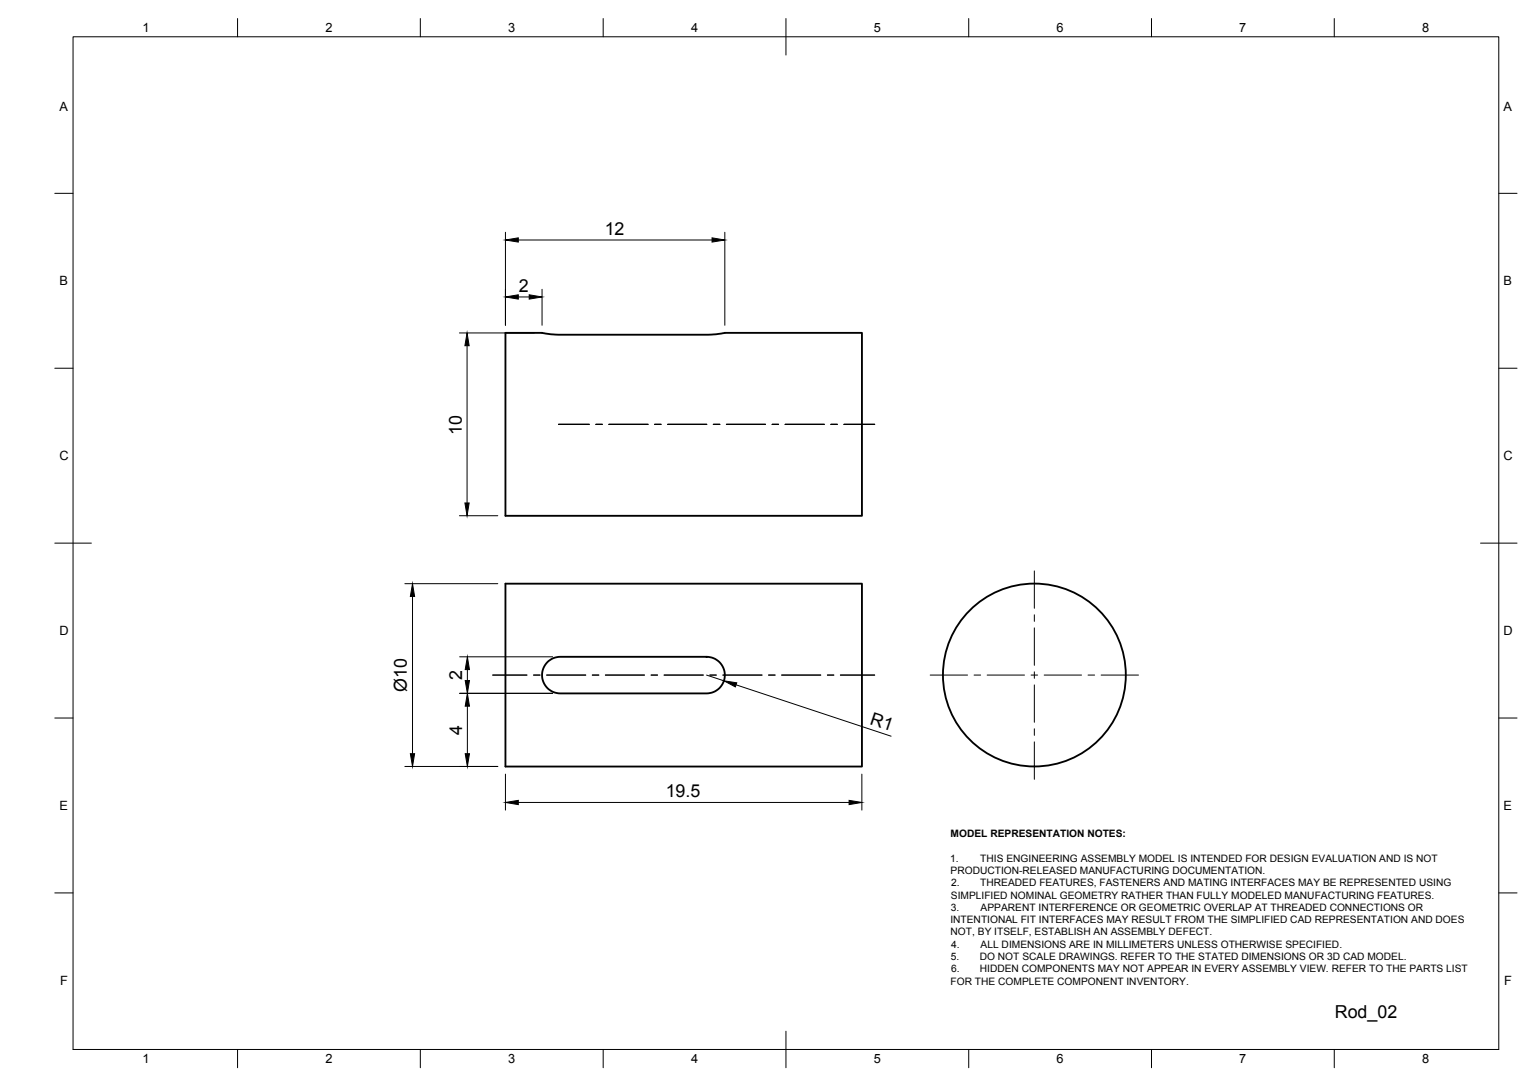
ISO-10303-21;
HEADER;
/* Generated by software containing ST-Developer
 * from STEP Tools, Inc. (www.steptools.com) 
 */

FILE_DESCRIPTION(
/* description */ (''),
/* implementation_level */ '2;1');

FILE_NAME(
/* name */ 'Rod_02.step',
/* time_stamp */ '2026-10-05T21:34:53-07:00',
/* author */ (''),
/* organization */ (''),
/* preprocessor_version */ 'ST-DEVELOPER v20.2',
/* originating_system */ 'Autodesk Translation Framework v15.15.0.0',
/* authorisation */ '');

FILE_SCHEMA (('AUTOMOTIVE_DESIGN { 1 0 10303 214 3 1 1 }'));
ENDSEC;

DATA;
#10=MECHANICAL_DESIGN_GEOMETRIC_PRESENTATION_REPRESENTATION('',(#71),#9822);
#53=SHAPE_REPRESENTATION_RELATIONSHIP('SRR','None',#9863,#62);
#62=ADVANCED_BREP_SHAPE_REPRESENTATION('',(#80),#9819);
#71=STYLED_ITEM('',(#9912),#80);
#80=MANIFOLD_SOLID_BREP('Body1',#3294);
#98=FACE_BOUND('',#637,.T.);
#155=B_SPLINE_CURVE_WITH_KNOTS('',3,(#9682,#9683,#9684,#9685,#9686,#9687,
#9688,#9689,#9690,#9691,#9692,#9693,#9694,#9695,#9696,#9697,#9698,#9699),
 .UNSPECIFIED.,.F.,.F.,(4,2,2,2,2,2,2,2,4),(-0.302227736861757,-0.264448211272738,
-0.226668685683718,-0.188891277057298,-0.151113868430879,-0.113336459804459,
-0.0755590511780388,-0.0377795255890194,0.),.UNSPECIFIED.);
#156=B_SPLINE_CURVE_WITH_KNOTS('',3,(#9712,#9713,#9714,#9715,#9716,#9717,
#9718,#9719,#9720,#9721,#9722,#9723,#9724,#9725,#9726,#9727,#9728,#9729),
 .UNSPECIFIED.,.F.,.F.,(4,2,2,2,2,2,2,2,4),(-0.604455473723515,-0.566675948134495,
-0.528896422545476,-0.491119013919056,-0.453341605292636,-0.415564196666216,
-0.377786788039796,-0.340007262450777,-0.302227736861757),.UNSPECIFIED.);
#252=PLANE('',#3684);
#253=PLANE('',#3687);
#254=PLANE('',#3689);
#255=PLANE('',#3691);
#256=PLANE('',#3695);
#430=FACE_OUTER_BOUND('',#630,.T.);
#431=FACE_OUTER_BOUND('',#631,.T.);
#432=FACE_OUTER_BOUND('',#632,.T.);
#433=FACE_OUTER_BOUND('',#633,.T.);
#434=FACE_OUTER_BOUND('',#634,.T.);
#435=FACE_OUTER_BOUND('',#635,.T.);
#436=FACE_OUTER_BOUND('',#636,.T.);
#437=FACE_OUTER_BOUND('',#638,.T.);
#630=EDGE_LOOP('',(#2948,#2949,#2950,#2951));
#631=EDGE_LOOP('',(#2952,#2953,#2954,#2955));
#632=EDGE_LOOP('',(#2956,#2957,#2958,#2959));
#633=EDGE_LOOP('',(#2960,#2961,#2962,#2963));
#634=EDGE_LOOP('',(#2964,#2965,#2966,#2967));
#635=EDGE_LOOP('',(#2968));
#636=EDGE_LOOP('',(#2969,#2970,#2971,#2972));
#637=EDGE_LOOP('',(#2973,#2974,#2975,#2976));
#638=EDGE_LOOP('',(#2977));
#885=LINE('',#9674,#1144);
#886=LINE('',#9676,#1145);
#887=LINE('',#9678,#1146);
#888=LINE('',#9679,#1147);
#889=LINE('',#9701,#1148);
#890=LINE('',#9705,#1149);
#891=LINE('',#9709,#1150);
#892=LINE('',#9710,#1151);
#893=LINE('',#9735,#1152);
#1144=VECTOR('',#4537,10.);
#1145=VECTOR('',#4538,10.);
#1146=VECTOR('',#4539,10.);
#1147=VECTOR('',#4540,10.);
#1148=VECTOR('',#4543,10.);
#1149=VECTOR('',#4548,10.);
#1150=VECTOR('',#4553,10.);
#1151=VECTOR('',#4554,10.);
#1152=VECTOR('',#4563,5.);
#1307=CIRCLE('',#3686,1.);
#1308=CIRCLE('',#3688,1.);
#1309=CIRCLE('',#3692,5.);
#1310=CIRCLE('',#3694,5.);
#1599=VERTEX_POINT('',#9672);
#1600=VERTEX_POINT('',#9673);
#1601=VERTEX_POINT('',#9675);
#1602=VERTEX_POINT('',#9677);
#1603=VERTEX_POINT('',#9681);
#1604=VERTEX_POINT('',#9700);
#1605=VERTEX_POINT('',#9704);
#1606=VERTEX_POINT('',#9708);
#1607=VERTEX_POINT('',#9731);
#1608=VERTEX_POINT('',#9734);
#2053=EDGE_CURVE('',#1599,#1600,#885,.T.);
#2054=EDGE_CURVE('',#1601,#1600,#886,.T.);
#2055=EDGE_CURVE('',#1601,#1602,#887,.T.);
#2056=EDGE_CURVE('',#1602,#1599,#888,.T.);
#2057=EDGE_CURVE('',#1600,#1603,#155,.T.);
#2058=EDGE_CURVE('',#1604,#1603,#889,.T.);
#2059=EDGE_CURVE('',#1604,#1601,#1307,.T.);
#2060=EDGE_CURVE('',#1605,#1604,#890,.T.);
#2061=EDGE_CURVE('',#1602,#1605,#1308,.T.);
#2062=EDGE_CURVE('',#1603,#1606,#891,.T.);
#2063=EDGE_CURVE('',#1605,#1606,#892,.T.);
#2064=EDGE_CURVE('',#1606,#1599,#156,.T.);
#2065=EDGE_CURVE('',#1607,#1607,#1309,.T.);
#2066=EDGE_CURVE('',#1607,#1608,#893,.T.);
#2067=EDGE_CURVE('',#1608,#1608,#1310,.T.);
#2948=ORIENTED_EDGE('',*,*,#2053,.T.);
#2949=ORIENTED_EDGE('',*,*,#2054,.F.);
#2950=ORIENTED_EDGE('',*,*,#2055,.T.);
#2951=ORIENTED_EDGE('',*,*,#2056,.T.);
#2952=ORIENTED_EDGE('',*,*,#2057,.T.);
#2953=ORIENTED_EDGE('',*,*,#2058,.F.);
#2954=ORIENTED_EDGE('',*,*,#2059,.T.);
#2955=ORIENTED_EDGE('',*,*,#2054,.T.);
#2956=ORIENTED_EDGE('',*,*,#2059,.F.);
#2957=ORIENTED_EDGE('',*,*,#2060,.F.);
#2958=ORIENTED_EDGE('',*,*,#2061,.F.);
#2959=ORIENTED_EDGE('',*,*,#2055,.F.);
#2960=ORIENTED_EDGE('',*,*,#2062,.T.);
#2961=ORIENTED_EDGE('',*,*,#2063,.F.);
#2962=ORIENTED_EDGE('',*,*,#2060,.T.);
#2963=ORIENTED_EDGE('',*,*,#2058,.T.);
#2964=ORIENTED_EDGE('',*,*,#2064,.T.);
#2965=ORIENTED_EDGE('',*,*,#2056,.F.);
#2966=ORIENTED_EDGE('',*,*,#2061,.T.);
#2967=ORIENTED_EDGE('',*,*,#2063,.T.);
#2968=ORIENTED_EDGE('',*,*,#2065,.F.);
#2969=ORIENTED_EDGE('',*,*,#2065,.T.);
#2970=ORIENTED_EDGE('',*,*,#2066,.T.);
#2971=ORIENTED_EDGE('',*,*,#2067,.T.);
#2972=ORIENTED_EDGE('',*,*,#2066,.F.);
#2973=ORIENTED_EDGE('',*,*,#2062,.F.);
#2974=ORIENTED_EDGE('',*,*,#2057,.F.);
#2975=ORIENTED_EDGE('',*,*,#2053,.F.);
#2976=ORIENTED_EDGE('',*,*,#2064,.F.);
#2977=ORIENTED_EDGE('',*,*,#2067,.F.);
#3096=CYLINDRICAL_SURFACE('',#3685,1.);
#3097=CYLINDRICAL_SURFACE('',#3690,1.);
#3098=CYLINDRICAL_SURFACE('',#3693,5.);
#3268=ADVANCED_FACE('',(#430),#252,.T.);
#3269=ADVANCED_FACE('',(#431),#3096,.F.);
#3270=ADVANCED_FACE('',(#432),#253,.T.);
#3271=ADVANCED_FACE('',(#433),#254,.T.);
#3272=ADVANCED_FACE('',(#434),#3097,.F.);
#3273=ADVANCED_FACE('',(#435),#255,.T.);
#3274=ADVANCED_FACE('',(#436,#98),#3098,.T.);
#3275=ADVANCED_FACE('',(#437),#256,.F.);
#3294=CLOSED_SHELL('',(#3268,#3269,#3270,#3271,#3272,#3273,#3274,#3275));
#3683=AXIS2_PLACEMENT_3D('',#9670,#4533,#4534);
#3684=AXIS2_PLACEMENT_3D('',#9671,#4535,#4536);
#3685=AXIS2_PLACEMENT_3D('',#9680,#4541,#4542);
#3686=AXIS2_PLACEMENT_3D('',#9702,#4544,#4545);
#3687=AXIS2_PLACEMENT_3D('',#9703,#4546,#4547);
#3688=AXIS2_PLACEMENT_3D('',#9706,#4549,#4550);
#3689=AXIS2_PLACEMENT_3D('',#9707,#4551,#4552);
#3690=AXIS2_PLACEMENT_3D('',#9711,#4555,#4556);
#3691=AXIS2_PLACEMENT_3D('',#9730,#4557,#4558);
#3692=AXIS2_PLACEMENT_3D('',#9732,#4559,#4560);
#3693=AXIS2_PLACEMENT_3D('',#9733,#4561,#4562);
#3694=AXIS2_PLACEMENT_3D('',#9736,#4564,#4565);
#3695=AXIS2_PLACEMENT_3D('',#9737,#4566,#4567);
#4533=DIRECTION('axis',(0.,0.,1.));
#4534=DIRECTION('refdir',(1.,0.,0.));
#4535=DIRECTION('center_axis',(-1.,0.,0.));
#4536=DIRECTION('ref_axis',(0.,0.,-1.));
#4537=DIRECTION('',(0.,0.,1.));
#4538=DIRECTION('',(0.,-1.,0.));
#4539=DIRECTION('',(0.,0.,-1.));
#4540=DIRECTION('',(0.,-1.,0.));
#4541=DIRECTION('center_axis',(0.,1.,0.));
#4542=DIRECTION('ref_axis',(1.,0.,0.));
#4543=DIRECTION('',(0.,-1.,0.));
#4544=DIRECTION('center_axis',(0.,1.,0.));
#4545=DIRECTION('ref_axis',(1.,0.,0.));
#4546=DIRECTION('center_axis',(0.,-1.,0.));
#4547=DIRECTION('ref_axis',(1.,0.,0.));
#4548=DIRECTION('',(0.,0.,1.));
#4549=DIRECTION('center_axis',(0.,1.,0.));
#4550=DIRECTION('ref_axis',(-1.,0.,0.));
#4551=DIRECTION('center_axis',(1.,0.,0.));
#4552=DIRECTION('ref_axis',(0.,0.,1.));
#4553=DIRECTION('',(0.,0.,-1.));
#4554=DIRECTION('',(0.,-1.,0.));
#4555=DIRECTION('center_axis',(0.,1.,0.));
#4556=DIRECTION('ref_axis',(-1.,0.,0.));
#4557=DIRECTION('center_axis',(0.,0.,1.));
#4558=DIRECTION('ref_axis',(-1.,0.,0.));
#4559=DIRECTION('center_axis',(0.,0.,-1.));
#4560=DIRECTION('ref_axis',(-1.,0.,0.));
#4561=DIRECTION('center_axis',(0.,0.,1.));
#4562=DIRECTION('ref_axis',(-1.,0.,0.));
#4563=DIRECTION('',(0.,0.,-1.));
#4564=DIRECTION('center_axis',(0.,0.,1.));
#4565=DIRECTION('ref_axis',(-1.,0.,0.));
#4566=DIRECTION('center_axis',(0.,0.,1.));
#4567=DIRECTION('ref_axis',(-1.,0.,0.));
#9670=CARTESIAN_POINT('',(0.,0.,0.));
#9671=CARTESIAN_POINT('Origin',(1.,0.,-6.5));
#9672=CARTESIAN_POINT('',(1.,-4.89897948556636,-14.5));
#9673=CARTESIAN_POINT('',(1.,-4.89897948556636,-6.5));
#9674=CARTESIAN_POINT('',(1.,-4.89897948556636,-12.));
#9675=CARTESIAN_POINT('',(1.,-4.,-6.5));
#9676=CARTESIAN_POINT('',(1.,0.,-6.5));
#9677=CARTESIAN_POINT('',(1.,-4.,-14.5));
#9678=CARTESIAN_POINT('',(1.,-4.,-8.5));
#9679=CARTESIAN_POINT('',(1.,0.,-14.5));
#9680=CARTESIAN_POINT('Origin',(0.,0.,-6.5));
#9681=CARTESIAN_POINT('',(-1.,-4.89897948556636,-6.5));
#9682=CARTESIAN_POINT('Ctrl Pts',(1.,-4.89897948556636,-6.5));
#9683=CARTESIAN_POINT('Ctrl Pts',(1.,-4.89897948556636,-6.3740682480366));
#9684=CARTESIAN_POINT('Ctrl Pts',(0.974762796248615,-4.90433876618447,-6.23998222283811));
#9685=CARTESIAN_POINT('Ctrl Pts',(0.872605417648384,-4.92354150792771,-5.99370799496995));
#9686=CARTESIAN_POINT('Ctrl Pts',(0.795703102192088,-4.93709085101933,-5.88148953981899));
#9687=CARTESIAN_POINT('Ctrl Pts',(0.618515424645094,-4.96240337638318,-5.704301862272));
#9688=CARTESIAN_POINT('Ctrl Pts',(0.506294861197626,-4.97583347151864,-5.62739565845524));
#9689=CARTESIAN_POINT('Ctrl Pts',(0.260013306081865,-4.99476188647081,-5.52523545776417));
#9690=CARTESIAN_POINT('Ctrl Pts',(0.125924695421399,-5.,-5.5));
#9691=CARTESIAN_POINT('Ctrl Pts',(-0.1259246954214,-5.,-5.5));
#9692=CARTESIAN_POINT('Ctrl Pts',(-0.260013306081865,-4.99476188647081,
-5.52523545776417));
#9693=CARTESIAN_POINT('Ctrl Pts',(-0.506294861197626,-4.97583347151864,
-5.62739565845524));
#9694=CARTESIAN_POINT('Ctrl Pts',(-0.618515424645094,-4.96240337638318,
-5.704301862272));
#9695=CARTESIAN_POINT('Ctrl Pts',(-0.795703102192089,-4.93709085101933,
-5.88148953981899));
#9696=CARTESIAN_POINT('Ctrl Pts',(-0.872605417648382,-4.92354150792771,
-5.99370799496995));
#9697=CARTESIAN_POINT('Ctrl Pts',(-0.974762796248614,-4.90433876618447,
-6.23998222283811));
#9698=CARTESIAN_POINT('Ctrl Pts',(-1.,-4.89897948556636,-6.3740682480366));
#9699=CARTESIAN_POINT('Ctrl Pts',(-1.,-4.89897948556636,-6.5));
#9700=CARTESIAN_POINT('',(-1.,-4.,-6.5));
#9701=CARTESIAN_POINT('',(-1.,0.,-6.5));
#9702=CARTESIAN_POINT('Origin',(0.,-4.,-6.5));
#9703=CARTESIAN_POINT('Origin',(0.,-4.,-10.5));
#9704=CARTESIAN_POINT('',(-1.,-4.,-14.5));
#9705=CARTESIAN_POINT('',(-1.,-4.,-12.5));
#9706=CARTESIAN_POINT('Origin',(0.,-4.,-14.5));
#9707=CARTESIAN_POINT('Origin',(-1.,0.,-14.5));
#9708=CARTESIAN_POINT('',(-1.,-4.89897948556636,-14.5));
#9709=CARTESIAN_POINT('',(-1.,-4.89897948556636,-12.));
#9710=CARTESIAN_POINT('',(-1.,0.,-14.5));
#9711=CARTESIAN_POINT('Origin',(0.,0.,-14.5));
#9712=CARTESIAN_POINT('Ctrl Pts',(-1.,-4.89897948556636,-14.5));
#9713=CARTESIAN_POINT('Ctrl Pts',(-1.,-4.89897948556636,-14.6259317519634));
#9714=CARTESIAN_POINT('Ctrl Pts',(-0.974762796248615,-4.90433876618447,
-14.7600177771619));
#9715=CARTESIAN_POINT('Ctrl Pts',(-0.872605417648385,-4.92354150792771,
-15.00629200503));
#9716=CARTESIAN_POINT('Ctrl Pts',(-0.795703102192088,-4.93709085101933,
-15.118510460181));
#9717=CARTESIAN_POINT('Ctrl Pts',(-0.618515424645093,-4.96240337638318,
-15.295698137728));
#9718=CARTESIAN_POINT('Ctrl Pts',(-0.506294861197626,-4.97583347151864,
-15.3726043415448));
#9719=CARTESIAN_POINT('Ctrl Pts',(-0.260013306081865,-4.99476188647081,
-15.4747645422358));
#9720=CARTESIAN_POINT('Ctrl Pts',(-0.125924695421399,-5.,-15.5));
#9721=CARTESIAN_POINT('Ctrl Pts',(0.1259246954214,-5.,-15.5));
#9722=CARTESIAN_POINT('Ctrl Pts',(0.260013306081866,-4.99476188647081,-15.4747645422358));
#9723=CARTESIAN_POINT('Ctrl Pts',(0.506294861197627,-4.97583347151864,-15.3726043415448));
#9724=CARTESIAN_POINT('Ctrl Pts',(0.618515424645094,-4.96240337638318,-15.295698137728));
#9725=CARTESIAN_POINT('Ctrl Pts',(0.795703102192089,-4.93709085101933,-15.118510460181));
#9726=CARTESIAN_POINT('Ctrl Pts',(0.872605417648382,-4.92354150792771,-15.0062920050301));
#9727=CARTESIAN_POINT('Ctrl Pts',(0.974762796248614,-4.90433876618447,-14.7600177771619));
#9728=CARTESIAN_POINT('Ctrl Pts',(1.,-4.89897948556636,-14.6259317519634));
#9729=CARTESIAN_POINT('Ctrl Pts',(1.,-4.89897948556636,-14.5));
#9730=CARTESIAN_POINT('Origin',(0.,0.,-3.5));
#9731=CARTESIAN_POINT('',(5.,6.12323399573677E-16,-3.5));
#9732=CARTESIAN_POINT('Origin',(0.,0.,-3.5));
#9733=CARTESIAN_POINT('Origin',(0.,0.,-12.));
#9734=CARTESIAN_POINT('',(5.,6.12323399573677E-16,-23.));
#9735=CARTESIAN_POINT('',(5.,6.12323399573677E-16,-12.));
#9736=CARTESIAN_POINT('Origin',(0.,0.,-23.));
#9737=CARTESIAN_POINT('Origin',(0.,0.,-23.));
#9808=UNCERTAINTY_MEASURE_WITH_UNIT(LENGTH_MEASURE(0.01),#9823,
'DISTANCE_ACCURACY_VALUE',
'Maximum model space distance between geometric entities at asserted c
onnectivities');
#9811=UNCERTAINTY_MEASURE_WITH_UNIT(LENGTH_MEASURE(0.01),#9823,
'DISTANCE_ACCURACY_VALUE',
'Maximum model space distance between geometric entities at asserted c
onnectivities');
#9819=(
GEOMETRIC_REPRESENTATION_CONTEXT(3)
GLOBAL_UNCERTAINTY_ASSIGNED_CONTEXT((#9808))
GLOBAL_UNIT_ASSIGNED_CONTEXT((#9823,#9825,#9826))
REPRESENTATION_CONTEXT('','3D')
);
#9822=(
GEOMETRIC_REPRESENTATION_CONTEXT(3)
GLOBAL_UNCERTAINTY_ASSIGNED_CONTEXT((#9811))
GLOBAL_UNIT_ASSIGNED_CONTEXT((#9823,#9825,#9826))
REPRESENTATION_CONTEXT('','3D')
);
#9823=(
LENGTH_UNIT()
NAMED_UNIT(*)
SI_UNIT(.MILLI.,.METRE.)
);
#9825=(
NAMED_UNIT(*)
PLANE_ANGLE_UNIT()
SI_UNIT($,.RADIAN.)
);
#9826=(
NAMED_UNIT(*)
SI_UNIT($,.STERADIAN.)
SOLID_ANGLE_UNIT()
);
#9834=SHAPE_DEFINITION_REPRESENTATION(#9844,#9863);
#9844=PRODUCT_DEFINITION_SHAPE('',$,#9874);
#9863=SHAPE_REPRESENTATION('',(#3683),#9819);
#9866=PRODUCT_DEFINITION_CONTEXT('part definition',#9898,'design');
#9874=PRODUCT_DEFINITION('Rod_02','Rod_02',#9884,#9866);
#9884=PRODUCT_DEFINITION_FORMATION('',$,#9907);
#9898=APPLICATION_CONTEXT(
'Core Data for Automotive Mechanical Design Process');
#9899=PRODUCT_CONTEXT('part definition',#9898,'mechanical');
#9907=PRODUCT('Rod_02','Rod_02',$,(#9899));
#9912=PRESENTATION_STYLE_ASSIGNMENT((#9915));
#9915=SURFACE_STYLE_USAGE(.BOTH.,#9918);
#9918=SURFACE_SIDE_STYLE('',(#9921));
#9921=SURFACE_STYLE_FILL_AREA(#9924);
#9924=FILL_AREA_STYLE('Opaque(233,233,233)',(#9927));
#9927=FILL_AREA_STYLE_COLOUR('Opaque(233,233,233)',#9930);
#9930=COLOUR_RGB('Opaque(233,233,233)', 0.40784314, 0.44705882, 0.49803922);
ENDSEC;
END-ISO-10303-21;
